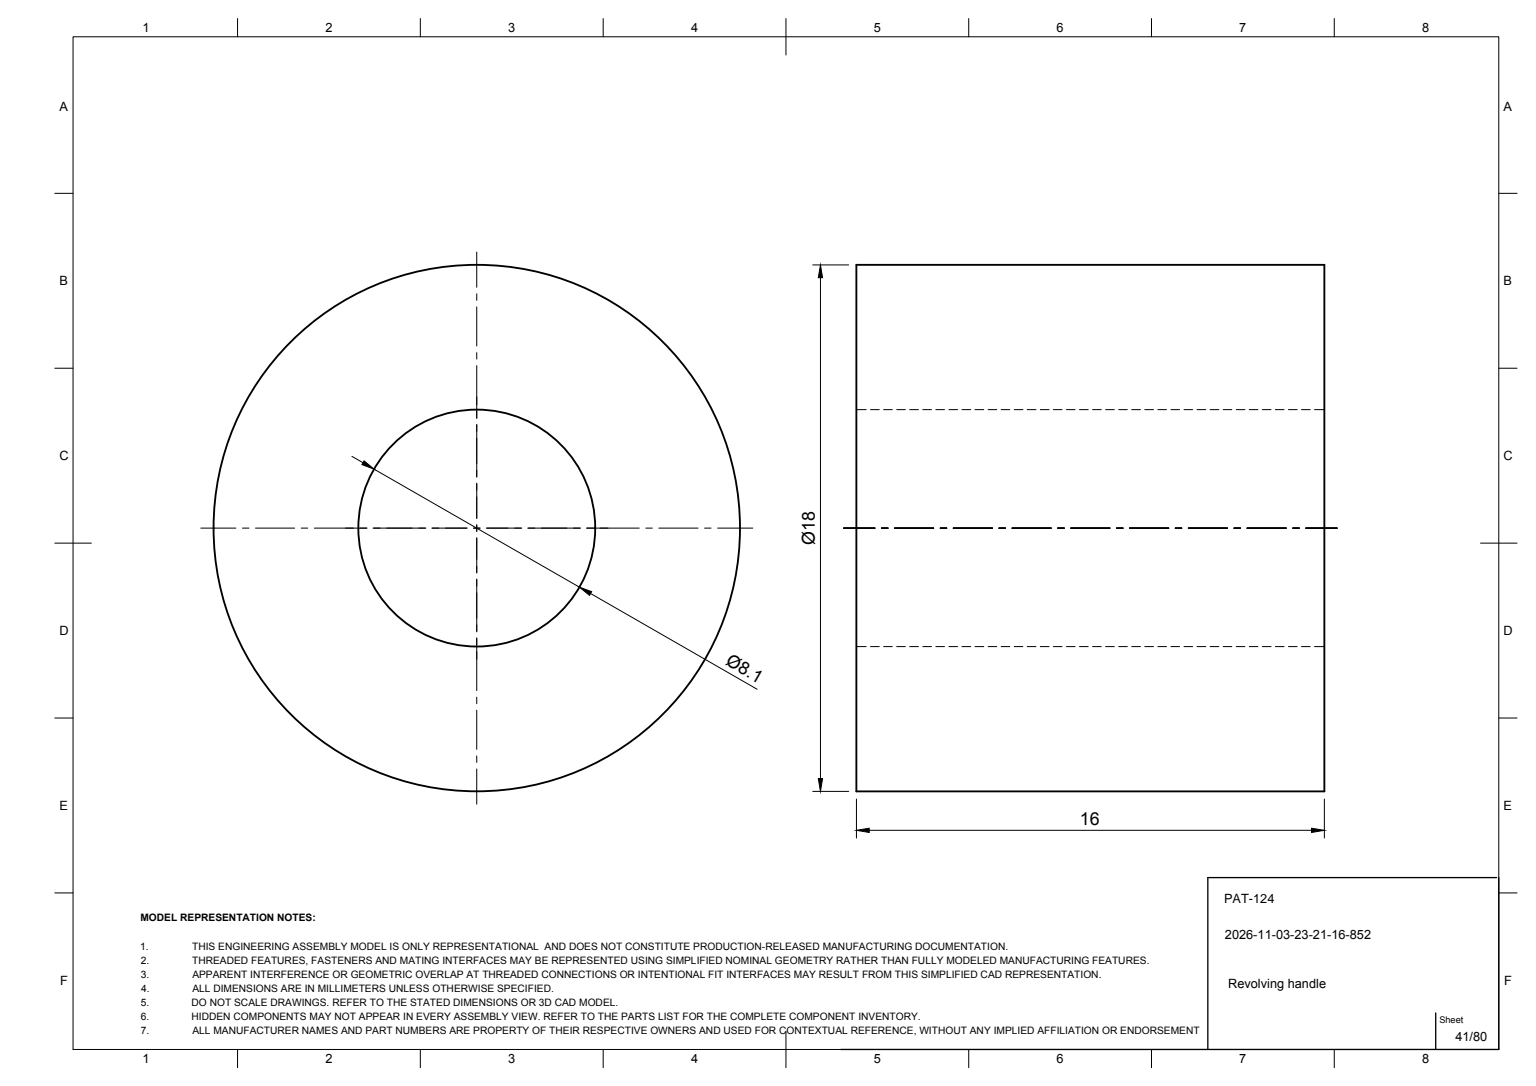
ISO-10303-21;
HEADER;
/* Generated by software containing ST-Developer
 * from STEP Tools, Inc. (www.steptools.com) 
 */

FILE_DESCRIPTION(
/* description */ ('XY cross-slide table'),
/* implementation_level */ '2;1');

FILE_NAME(
/* name */ 'Revolving handle.step',
/* time_stamp */ '2026-10-28T03:22:46-07:00',
/* author */ (''),
/* organization */ (''),
/* preprocessor_version */ 'ST-DEVELOPER v20.2',
/* originating_system */ 'Autodesk Translation Framework v15.17.0.0',
/* authorisation */ '');

FILE_SCHEMA (('AUTOMOTIVE_DESIGN { 1 0 10303 214 3 1 1 }'));
ENDSEC;

DATA;
#10=MECHANICAL_DESIGN_GEOMETRIC_PRESENTATION_REPRESENTATION('',(#1722),#62984);
#1541=SHAPE_REPRESENTATION_RELATIONSHIP('SRR','None',#63394,#1624);
#1624=ADVANCED_BREP_SHAPE_REPRESENTATION('',(#1832),#62931);
#1722=STYLED_ITEM('',(#63905),#1832);
#1832=MANIFOLD_SOLID_BREP('Body1',#23019);
#2079=FACE_BOUND('',#4974,.T.);
#2080=FACE_BOUND('',#4976,.T.);
#2543=PLANE('',#25088);
#2544=PLANE('',#25089);
#3465=FACE_OUTER_BOUND('',#4971,.T.);
#3466=FACE_OUTER_BOUND('',#4972,.T.);
#3467=FACE_OUTER_BOUND('',#4973,.T.);
#3468=FACE_OUTER_BOUND('',#4975,.T.);
#4971=EDGE_LOOP('',(#17744,#17745,#17746,#17747));
#4972=EDGE_LOOP('',(#17748,#17749,#17750,#17751));
#4973=EDGE_LOOP('',(#17752));
#4974=EDGE_LOOP('',(#17753));
#4975=EDGE_LOOP('',(#17754));
#4976=EDGE_LOOP('',(#17755));
#6571=LINE('',#47532,#8058);
#6572=LINE('',#47538,#8059);
#8058=VECTOR('',#29294,0.405);
#8059=VECTOR('',#29301,0.9);
#9291=CIRCLE('',#25083,0.405);
#9292=CIRCLE('',#25084,0.405);
#9293=CIRCLE('',#25086,0.9);
#9294=CIRCLE('',#25087,0.9);
#10731=VERTEX_POINT('',#47529);
#10732=VERTEX_POINT('',#47531);
#10733=VERTEX_POINT('',#47535);
#10734=VERTEX_POINT('',#47537);
#13256=EDGE_CURVE('',#10731,#10731,#9291,.T.);
#13257=EDGE_CURVE('',#10731,#10732,#6571,.T.);
#13258=EDGE_CURVE('',#10732,#10732,#9292,.T.);
#13259=EDGE_CURVE('',#10733,#10733,#9293,.T.);
#13260=EDGE_CURVE('',#10733,#10734,#6572,.T.);
#13261=EDGE_CURVE('',#10734,#10734,#9294,.T.);
#17744=ORIENTED_EDGE('',*,*,#13256,.F.);
#17745=ORIENTED_EDGE('',*,*,#13257,.T.);
#17746=ORIENTED_EDGE('',*,*,#13258,.T.);
#17747=ORIENTED_EDGE('',*,*,#13257,.F.);
#17748=ORIENTED_EDGE('',*,*,#13259,.F.);
#17749=ORIENTED_EDGE('',*,*,#13260,.T.);
#17750=ORIENTED_EDGE('',*,*,#13261,.T.);
#17751=ORIENTED_EDGE('',*,*,#13260,.F.);
#17752=ORIENTED_EDGE('',*,*,#13259,.T.);
#17753=ORIENTED_EDGE('',*,*,#13256,.T.);
#17754=ORIENTED_EDGE('',*,*,#13261,.F.);
#17755=ORIENTED_EDGE('',*,*,#13258,.F.);
#21331=CYLINDRICAL_SURFACE('',#25082,0.405);
#21332=CYLINDRICAL_SURFACE('',#25085,0.9);
#22246=ADVANCED_FACE('',(#3465),#21331,.F.);
#22247=ADVANCED_FACE('',(#3466),#21332,.T.);
#22248=ADVANCED_FACE('',(#3467,#2079),#2543,.T.);
#22249=ADVANCED_FACE('',(#3468,#2080),#2544,.F.);
#23019=CLOSED_SHELL('',(#22246,#22247,#22248,#22249));
#25081=AXIS2_PLACEMENT_3D('',#47527,#29288,#29289);
#25082=AXIS2_PLACEMENT_3D('',#47528,#29290,#29291);
#25083=AXIS2_PLACEMENT_3D('',#47530,#29292,#29293);
#25084=AXIS2_PLACEMENT_3D('',#47533,#29295,#29296);
#25085=AXIS2_PLACEMENT_3D('',#47534,#29297,#29298);
#25086=AXIS2_PLACEMENT_3D('',#47536,#29299,#29300);
#25087=AXIS2_PLACEMENT_3D('',#47539,#29302,#29303);
#25088=AXIS2_PLACEMENT_3D('',#47540,#29304,#29305);
#25089=AXIS2_PLACEMENT_3D('',#47541,#29306,#29307);
#29288=DIRECTION('axis',(0.,0.,1.));
#29289=DIRECTION('refdir',(1.,0.,0.));
#29290=DIRECTION('center_axis',(1.,0.,0.));
#29291=DIRECTION('ref_axis',(0.,0.,-1.));
#29292=DIRECTION('center_axis',(-1.,0.,0.));
#29293=DIRECTION('ref_axis',(0.,0.,-1.));
#29294=DIRECTION('',(-1.,0.,0.));
#29295=DIRECTION('center_axis',(-1.,0.,0.));
#29296=DIRECTION('ref_axis',(0.,0.,-1.));
#29297=DIRECTION('center_axis',(1.,0.,0.));
#29298=DIRECTION('ref_axis',(0.,0.,-1.));
#29299=DIRECTION('center_axis',(1.,0.,0.));
#29300=DIRECTION('ref_axis',(0.,0.,-1.));
#29301=DIRECTION('',(-1.,0.,0.));
#29302=DIRECTION('center_axis',(1.,0.,0.));
#29303=DIRECTION('ref_axis',(0.,0.,-1.));
#29304=DIRECTION('center_axis',(1.,0.,0.));
#29305=DIRECTION('ref_axis',(0.,0.,-1.));
#29306=DIRECTION('center_axis',(1.,0.,0.));
#29307=DIRECTION('ref_axis',(0.,0.,-1.));
#47527=CARTESIAN_POINT('',(0.,0.,0.));
#47528=CARTESIAN_POINT('Origin',(29.4,0.,6.5));
#47529=CARTESIAN_POINT('',(31.,-4.95981953654678E-17,6.905));
#47530=CARTESIAN_POINT('Origin',(31.,0.,6.5));
#47531=CARTESIAN_POINT('',(29.4,-4.95981953654678E-17,6.905));
#47532=CARTESIAN_POINT('',(29.4,-4.95981953654678E-17,6.905));
#47533=CARTESIAN_POINT('Origin',(29.4,0.,6.5));
#47534=CARTESIAN_POINT('Origin',(29.4,0.,6.5));
#47535=CARTESIAN_POINT('',(31.,-1.10218211923262E-16,7.4));
#47536=CARTESIAN_POINT('Origin',(31.,0.,6.5));
#47537=CARTESIAN_POINT('',(29.4,-1.10218211923262E-16,7.4));
#47538=CARTESIAN_POINT('',(29.4,-1.10218211923262E-16,7.4));
#47539=CARTESIAN_POINT('Origin',(29.4,0.,6.5));
#47540=CARTESIAN_POINT('Origin',(31.,0.,6.5));
#47541=CARTESIAN_POINT('Origin',(29.4,0.,6.5));
#62832=UNCERTAINTY_MEASURE_WITH_UNIT(LENGTH_MEASURE(0.001),#62985,
'DISTANCE_ACCURACY_VALUE',
'Maximum model space distance between geometric entities at asserted c
onnectivities');
#62885=UNCERTAINTY_MEASURE_WITH_UNIT(LENGTH_MEASURE(0.001),#62985,
'DISTANCE_ACCURACY_VALUE',
'Maximum model space distance between geometric entities at asserted c
onnectivities');
#62931=(
GEOMETRIC_REPRESENTATION_CONTEXT(3)
GLOBAL_UNCERTAINTY_ASSIGNED_CONTEXT((#62832))
GLOBAL_UNIT_ASSIGNED_CONTEXT((#62985,#62987,#62988))
REPRESENTATION_CONTEXT('','3D')
);
#62984=(
GEOMETRIC_REPRESENTATION_CONTEXT(3)
GLOBAL_UNCERTAINTY_ASSIGNED_CONTEXT((#62885))
GLOBAL_UNIT_ASSIGNED_CONTEXT((#62985,#62987,#62988))
REPRESENTATION_CONTEXT('','3D')
);
#62985=(
LENGTH_UNIT()
NAMED_UNIT(*)
SI_UNIT(.CENTI.,.METRE.)
);
#62987=(
NAMED_UNIT(*)
PLANE_ANGLE_UNIT()
SI_UNIT($,.RADIAN.)
);
#62988=(
NAMED_UNIT(*)
SI_UNIT($,.STERADIAN.)
SOLID_ANGLE_UNIT()
);
#63034=SHAPE_DEFINITION_REPRESENTATION(#63165,#63394);
#63165=PRODUCT_DEFINITION_SHAPE('',$,#63493);
#63394=SHAPE_REPRESENTATION('',(#25081),#62931);
#63447=PRODUCT_DEFINITION_CONTEXT('part definition',#63743,'design');
#63493=PRODUCT_DEFINITION('Revolving handle','Revolving handle',#63591,
#63447);
#63591=PRODUCT_DEFINITION_FORMATION('',$,#63790);
#63743=APPLICATION_CONTEXT(
'Core Data for Automotive Mechanical Design Process');
#63744=PRODUCT_CONTEXT('part definition',#63743,'mechanical');
#63790=PRODUCT('Revolving handle','Revolving handle','Revolving handle',
(#63744));
#63899=COLOUR_RGB('Sky Blue',0.24,0.69,0.87);
#63900=FILL_AREA_STYLE_COLOUR('',#63899);
#63901=FILL_AREA_STYLE('',(#63900));
#63902=SURFACE_STYLE_FILL_AREA(#63901);
#63903=SURFACE_SIDE_STYLE('',(#63902));
#63904=SURFACE_STYLE_USAGE(.BOTH.,#63903);
#63905=PRESENTATION_STYLE_ASSIGNMENT((#63904));
ENDSEC;
END-ISO-10303-21;
